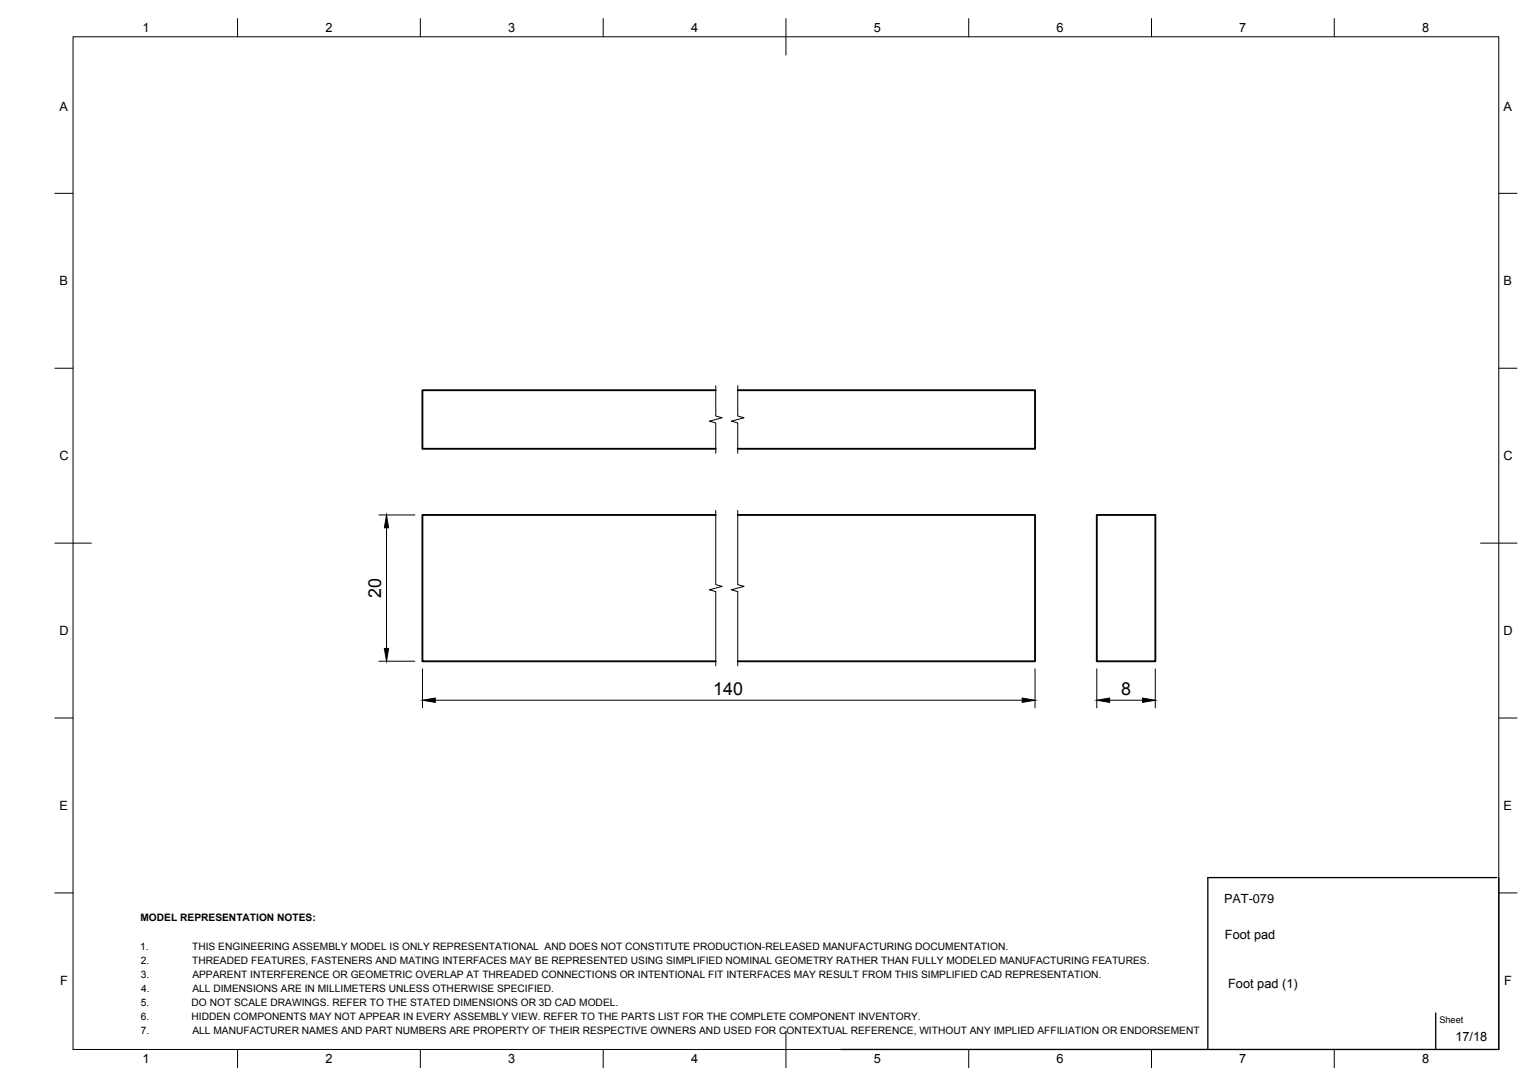
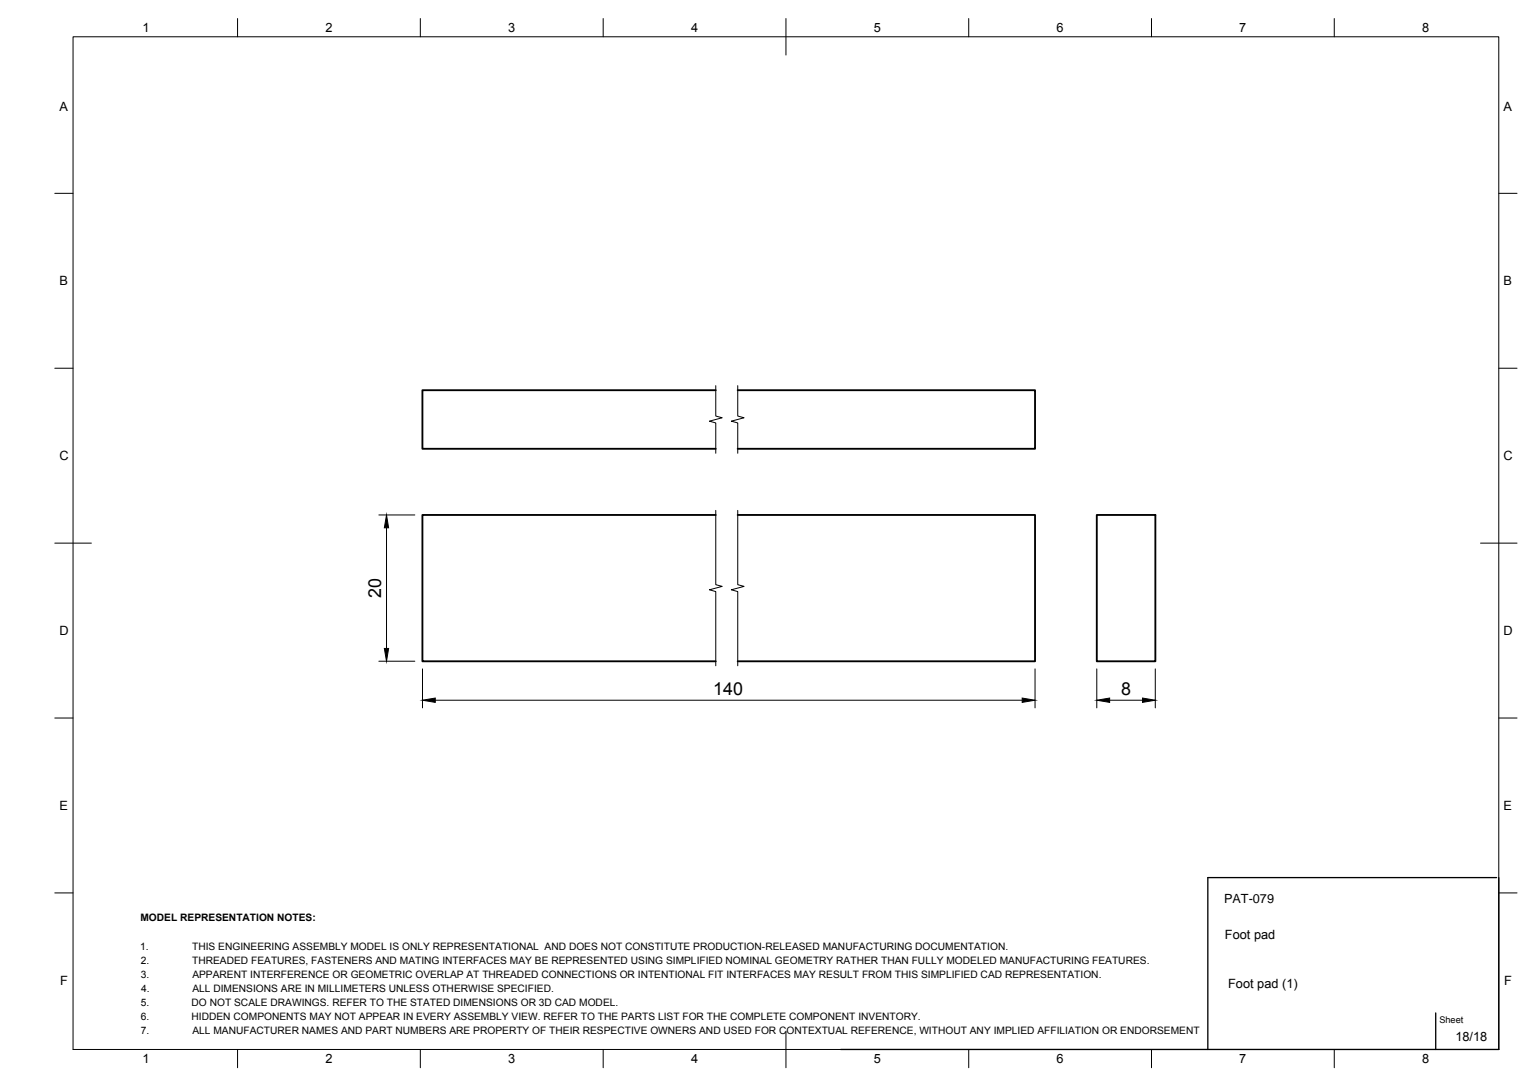
ISO-10303-21;
HEADER;
/* Generated by software containing ST-Developer
 * from STEP Tools, Inc. (www.steptools.com) 
 */

FILE_DESCRIPTION(
/* description */ ('Pipe clamp stand with threaded column'),
/* implementation_level */ '2;1');

FILE_NAME(
/* name */ 'Foot pad.step',
/* time_stamp */ '2026-10-27T10:55:48-07:00',
/* author */ (''),
/* organization */ (''),
/* preprocessor_version */ 'ST-DEVELOPER v20.2',
/* originating_system */ 'Autodesk Translation Framework v15.17.0.0',
/* authorisation */ '');

FILE_SCHEMA (('AUTOMOTIVE_DESIGN { 1 0 10303 214 3 1 1 }'));
ENDSEC;

DATA;
#10=MECHANICAL_DESIGN_GEOMETRIC_PRESENTATION_REPRESENTATION('',(#761),#34433);
#709=SHAPE_REPRESENTATION_RELATIONSHIP('SRR','None',#34551,#731);
#731=ADVANCED_BREP_SHAPE_REPRESENTATION('',(#791),#34419);
#761=STYLED_ITEM('',(#34736),#791);
#791=MANIFOLD_SOLID_BREP('Body1',#8788);
#967=PLANE('',#9496);
#968=PLANE('',#9497);
#969=PLANE('',#9498);
#970=PLANE('',#9499);
#971=PLANE('',#9500);
#972=PLANE('',#9501);
#1390=FACE_OUTER_BOUND('',#1920,.T.);
#1391=FACE_OUTER_BOUND('',#1921,.T.);
#1392=FACE_OUTER_BOUND('',#1922,.T.);
#1393=FACE_OUTER_BOUND('',#1923,.T.);
#1394=FACE_OUTER_BOUND('',#1924,.T.);
#1395=FACE_OUTER_BOUND('',#1925,.T.);
#1920=EDGE_LOOP('',(#7331,#7332,#7333,#7334));
#1921=EDGE_LOOP('',(#7335,#7336,#7337,#7338));
#1922=EDGE_LOOP('',(#7339,#7340,#7341,#7342));
#1923=EDGE_LOOP('',(#7343,#7344,#7345,#7346));
#1924=EDGE_LOOP('',(#7347,#7348,#7349,#7350));
#1925=EDGE_LOOP('',(#7351,#7352,#7353,#7354));
#2507=LINE('',#28628,#3124);
#2508=LINE('',#28630,#3125);
#2509=LINE('',#28632,#3126);
#2510=LINE('',#28633,#3127);
#2511=LINE('',#28636,#3128);
#2512=LINE('',#28638,#3129);
#2513=LINE('',#28639,#3130);
#2514=LINE('',#28642,#3131);
#2515=LINE('',#28644,#3132);
#2516=LINE('',#28645,#3133);
#2517=LINE('',#28647,#3134);
#2518=LINE('',#28648,#3135);
#3124=VECTOR('',#11064,1.);
#3125=VECTOR('',#11065,1.);
#3126=VECTOR('',#11066,1.);
#3127=VECTOR('',#11067,1.);
#3128=VECTOR('',#11070,1.);
#3129=VECTOR('',#11071,1.);
#3130=VECTOR('',#11072,1.);
#3131=VECTOR('',#11075,1.);
#3132=VECTOR('',#11076,1.);
#3133=VECTOR('',#11077,1.);
#3134=VECTOR('',#11080,1.);
#3135=VECTOR('',#11081,1.);
#4050=VERTEX_POINT('',#28626);
#4051=VERTEX_POINT('',#28627);
#4052=VERTEX_POINT('',#28629);
#4053=VERTEX_POINT('',#28631);
#4054=VERTEX_POINT('',#28635);
#4055=VERTEX_POINT('',#28637);
#4056=VERTEX_POINT('',#28641);
#4057=VERTEX_POINT('',#28643);
#5179=EDGE_CURVE('',#4050,#4051,#2507,.T.);
#5180=EDGE_CURVE('',#4051,#4052,#2508,.T.);
#5181=EDGE_CURVE('',#4053,#4052,#2509,.T.);
#5182=EDGE_CURVE('',#4050,#4053,#2510,.T.);
#5183=EDGE_CURVE('',#4054,#4050,#2511,.T.);
#5184=EDGE_CURVE('',#4055,#4053,#2512,.T.);
#5185=EDGE_CURVE('',#4054,#4055,#2513,.T.);
#5186=EDGE_CURVE('',#4056,#4054,#2514,.T.);
#5187=EDGE_CURVE('',#4057,#4055,#2515,.T.);
#5188=EDGE_CURVE('',#4056,#4057,#2516,.T.);
#5189=EDGE_CURVE('',#4051,#4056,#2517,.T.);
#5190=EDGE_CURVE('',#4052,#4057,#2518,.T.);
#7331=ORIENTED_EDGE('',*,*,#5179,.T.);
#7332=ORIENTED_EDGE('',*,*,#5180,.T.);
#7333=ORIENTED_EDGE('',*,*,#5181,.F.);
#7334=ORIENTED_EDGE('',*,*,#5182,.F.);
#7335=ORIENTED_EDGE('',*,*,#5183,.T.);
#7336=ORIENTED_EDGE('',*,*,#5182,.T.);
#7337=ORIENTED_EDGE('',*,*,#5184,.F.);
#7338=ORIENTED_EDGE('',*,*,#5185,.F.);
#7339=ORIENTED_EDGE('',*,*,#5186,.T.);
#7340=ORIENTED_EDGE('',*,*,#5185,.T.);
#7341=ORIENTED_EDGE('',*,*,#5187,.F.);
#7342=ORIENTED_EDGE('',*,*,#5188,.F.);
#7343=ORIENTED_EDGE('',*,*,#5189,.T.);
#7344=ORIENTED_EDGE('',*,*,#5188,.T.);
#7345=ORIENTED_EDGE('',*,*,#5190,.F.);
#7346=ORIENTED_EDGE('',*,*,#5180,.F.);
#7347=ORIENTED_EDGE('',*,*,#5190,.T.);
#7348=ORIENTED_EDGE('',*,*,#5187,.T.);
#7349=ORIENTED_EDGE('',*,*,#5184,.T.);
#7350=ORIENTED_EDGE('',*,*,#5181,.T.);
#7351=ORIENTED_EDGE('',*,*,#5189,.F.);
#7352=ORIENTED_EDGE('',*,*,#5179,.F.);
#7353=ORIENTED_EDGE('',*,*,#5183,.F.);
#7354=ORIENTED_EDGE('',*,*,#5186,.F.);
#8627=ADVANCED_FACE('',(#1390),#967,.T.);
#8628=ADVANCED_FACE('',(#1391),#968,.T.);
#8629=ADVANCED_FACE('',(#1392),#969,.T.);
#8630=ADVANCED_FACE('',(#1393),#970,.T.);
#8631=ADVANCED_FACE('',(#1394),#971,.T.);
#8632=ADVANCED_FACE('',(#1395),#972,.F.);
#8788=CLOSED_SHELL('',(#8627,#8628,#8629,#8630,#8631,#8632));
#9495=AXIS2_PLACEMENT_3D('',#28624,#11060,#11061);
#9496=AXIS2_PLACEMENT_3D('',#28625,#11062,#11063);
#9497=AXIS2_PLACEMENT_3D('',#28634,#11068,#11069);
#9498=AXIS2_PLACEMENT_3D('',#28640,#11073,#11074);
#9499=AXIS2_PLACEMENT_3D('',#28646,#11078,#11079);
#9500=AXIS2_PLACEMENT_3D('',#28649,#11082,#11083);
#9501=AXIS2_PLACEMENT_3D('',#28650,#11084,#11085);
#11060=DIRECTION('axis',(0.,0.,1.));
#11061=DIRECTION('refdir',(1.,0.,0.));
#11062=DIRECTION('center_axis',(0.,1.,0.));
#11063=DIRECTION('ref_axis',(-1.,0.,0.));
#11064=DIRECTION('',(-1.,0.,0.));
#11065=DIRECTION('',(0.,0.,1.));
#11066=DIRECTION('',(-1.,0.,0.));
#11067=DIRECTION('',(0.,0.,1.));
#11068=DIRECTION('center_axis',(1.,0.,0.));
#11069=DIRECTION('ref_axis',(0.,1.,0.));
#11070=DIRECTION('',(0.,1.,0.));
#11071=DIRECTION('',(0.,1.,0.));
#11072=DIRECTION('',(0.,0.,1.));
#11073=DIRECTION('center_axis',(0.,-1.,0.));
#11074=DIRECTION('ref_axis',(1.,0.,0.));
#11075=DIRECTION('',(1.,0.,0.));
#11076=DIRECTION('',(1.,0.,0.));
#11077=DIRECTION('',(0.,0.,1.));
#11078=DIRECTION('center_axis',(-1.,0.,0.));
#11079=DIRECTION('ref_axis',(0.,-1.,0.));
#11080=DIRECTION('',(0.,-1.,0.));
#11081=DIRECTION('',(0.,-1.,0.));
#11082=DIRECTION('center_axis',(0.,0.,1.));
#11083=DIRECTION('ref_axis',(1.,0.,0.));
#11084=DIRECTION('center_axis',(0.,0.,1.));
#11085=DIRECTION('ref_axis',(1.,0.,0.));
#28624=CARTESIAN_POINT('',(0.,0.,0.));
#28625=CARTESIAN_POINT('Origin',(-11.5,7.,-0.8));
#28626=CARTESIAN_POINT('',(-11.5,7.,-0.8));
#28627=CARTESIAN_POINT('',(-13.5,7.,-0.8));
#28628=CARTESIAN_POINT('',(-11.5,7.,-0.8));
#28629=CARTESIAN_POINT('',(-13.5,7.,0.));
#28630=CARTESIAN_POINT('',(-13.5,7.,-0.8));
#28631=CARTESIAN_POINT('',(-11.5,7.,0.));
#28632=CARTESIAN_POINT('',(-11.5,7.,0.));
#28633=CARTESIAN_POINT('',(-11.5,7.,-0.8));
#28634=CARTESIAN_POINT('Origin',(-11.5,-7.,-0.8));
#28635=CARTESIAN_POINT('',(-11.5,-7.,-0.8));
#28636=CARTESIAN_POINT('',(-11.5,-7.,-0.8));
#28637=CARTESIAN_POINT('',(-11.5,-7.,0.));
#28638=CARTESIAN_POINT('',(-11.5,-7.,0.));
#28639=CARTESIAN_POINT('',(-11.5,-7.,-0.8));
#28640=CARTESIAN_POINT('Origin',(-13.5,-7.,-0.8));
#28641=CARTESIAN_POINT('',(-13.5,-7.,-0.8));
#28642=CARTESIAN_POINT('',(-13.5,-7.,-0.8));
#28643=CARTESIAN_POINT('',(-13.5,-7.,0.));
#28644=CARTESIAN_POINT('',(-13.5,-7.,0.));
#28645=CARTESIAN_POINT('',(-13.5,-7.,-0.8));
#28646=CARTESIAN_POINT('Origin',(-13.5,7.,-0.8));
#28647=CARTESIAN_POINT('',(-13.5,7.,-0.8));
#28648=CARTESIAN_POINT('',(-13.5,7.,0.));
#28649=CARTESIAN_POINT('Origin',(-12.5,0.,0.));
#28650=CARTESIAN_POINT('Origin',(-12.5,0.,-0.8));
#34390=UNCERTAINTY_MEASURE_WITH_UNIT(LENGTH_MEASURE(0.001),#34434,
'DISTANCE_ACCURACY_VALUE',
'Maximum model space distance between geometric entities at asserted c
onnectivities');
#34404=UNCERTAINTY_MEASURE_WITH_UNIT(LENGTH_MEASURE(0.001),#34434,
'DISTANCE_ACCURACY_VALUE',
'Maximum model space distance between geometric entities at asserted c
onnectivities');
#34419=(
GEOMETRIC_REPRESENTATION_CONTEXT(3)
GLOBAL_UNCERTAINTY_ASSIGNED_CONTEXT((#34390))
GLOBAL_UNIT_ASSIGNED_CONTEXT((#34434,#34436,#34437))
REPRESENTATION_CONTEXT('','3D')
);
#34433=(
GEOMETRIC_REPRESENTATION_CONTEXT(3)
GLOBAL_UNCERTAINTY_ASSIGNED_CONTEXT((#34404))
GLOBAL_UNIT_ASSIGNED_CONTEXT((#34434,#34436,#34437))
REPRESENTATION_CONTEXT('','3D')
);
#34434=(
LENGTH_UNIT()
NAMED_UNIT(*)
SI_UNIT(.CENTI.,.METRE.)
);
#34436=(
NAMED_UNIT(*)
PLANE_ANGLE_UNIT()
SI_UNIT($,.RADIAN.)
);
#34437=(
NAMED_UNIT(*)
SI_UNIT($,.STERADIAN.)
SOLID_ANGLE_UNIT()
);
#34452=SHAPE_DEFINITION_REPRESENTATION(#34480,#34551);
#34480=PRODUCT_DEFINITION_SHAPE('',$,#34580);
#34551=SHAPE_REPRESENTATION('',(#9495),#34419);
#34565=PRODUCT_DEFINITION_CONTEXT('part definition',#34651,'design');
#34580=PRODUCT_DEFINITION('Foot pad','Foot pad',#34608,#34565);
#34608=PRODUCT_DEFINITION_FORMATION('',$,#34667);
#34651=APPLICATION_CONTEXT(
'Core Data for Automotive Mechanical Design Process');
#34652=PRODUCT_CONTEXT('part definition',#34651,'mechanical');
#34667=PRODUCT('Foot pad','Foot pad','Foot pad',(#34652));
#34730=COLOUR_RGB('Sky Blue',0.24,0.69,0.87);
#34731=FILL_AREA_STYLE_COLOUR('',#34730);
#34732=FILL_AREA_STYLE('',(#34731));
#34733=SURFACE_STYLE_FILL_AREA(#34732);
#34734=SURFACE_SIDE_STYLE('',(#34733));
#34735=SURFACE_STYLE_USAGE(.BOTH.,#34734);
#34736=PRESENTATION_STYLE_ASSIGNMENT((#34735));
ENDSEC;
END-ISO-10303-21;
